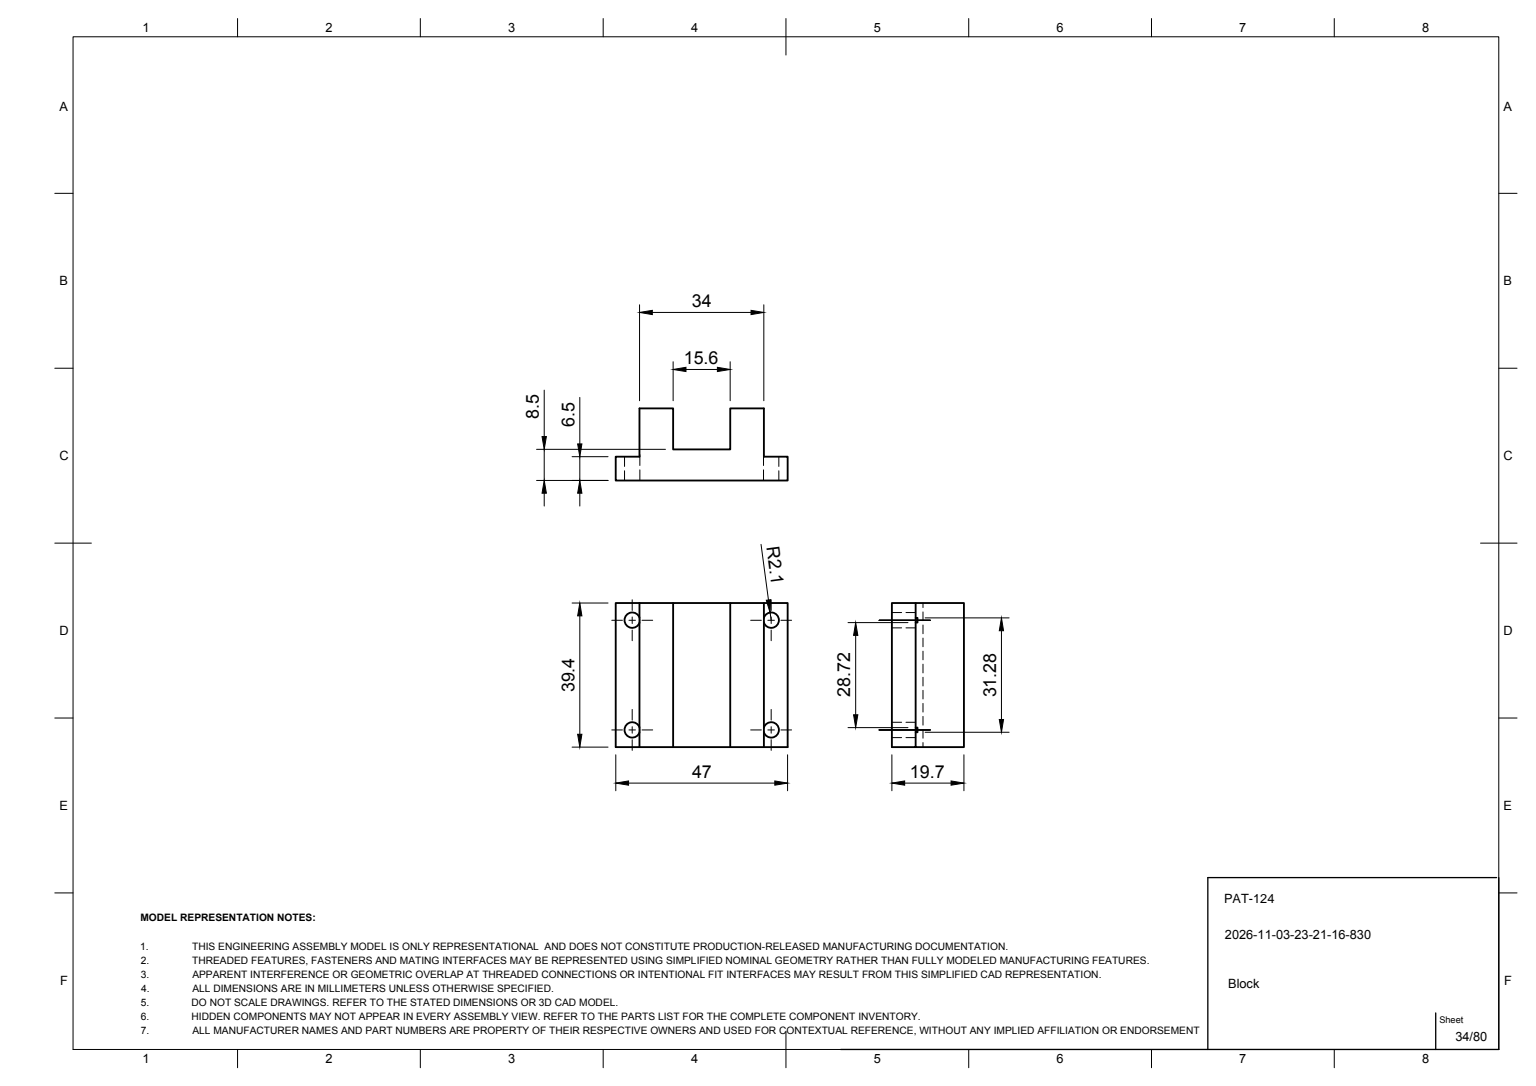
ISO-10303-21;
HEADER;
/* Generated by software containing ST-Developer
 * from STEP Tools, Inc. (www.steptools.com) 
 */

FILE_DESCRIPTION(
/* description */ ('XY cross-slide table'),
/* implementation_level */ '2;1');

FILE_NAME(
/* name */ 'Block.step',
/* time_stamp */ '2026-10-28T03:22:46-07:00',
/* author */ (''),
/* organization */ (''),
/* preprocessor_version */ 'ST-DEVELOPER v20.2',
/* originating_system */ 'Autodesk Translation Framework v15.17.0.0',
/* authorisation */ '');

FILE_SCHEMA (('AUTOMOTIVE_DESIGN { 1 0 10303 214 3 1 1 }'));
ENDSEC;

DATA;
#10=MECHANICAL_DESIGN_GEOMETRIC_PRESENTATION_REPRESENTATION('',(#1709),#62984);
#1528=SHAPE_REPRESENTATION_RELATIONSHIP('SRR','None',#63380,#1611);
#1611=ADVANCED_BREP_SHAPE_REPRESENTATION('',(#1822),#62917);
#1709=STYLED_ITEM('',(#63891),#1822);
#1822=MANIFOLD_SOLID_BREP('Body1',#23003);
#2042=FACE_BOUND('',#4647,.T.);
#2043=FACE_BOUND('',#4648,.T.);
#2044=FACE_BOUND('',#4649,.T.);
#2045=FACE_BOUND('',#4650,.T.);
#2439=PLANE('',#24650);
#2440=PLANE('',#24656);
#2441=PLANE('',#24662);
#2442=PLANE('',#24668);
#2443=PLANE('',#24674);
#2444=PLANE('',#24675);
#2445=PLANE('',#24676);
#2446=PLANE('',#24677);
#2447=PLANE('',#24678);
#2448=PLANE('',#24679);
#2449=PLANE('',#24680);
#2450=PLANE('',#24681);
#2451=PLANE('',#24682);
#2452=PLANE('',#24683);
#2453=PLANE('',#24684);
#2454=PLANE('',#24685);
#2455=PLANE('',#24686);
#2456=PLANE('',#24687);
#3164=FACE_OUTER_BOUND('',#4633,.T.);
#3165=FACE_OUTER_BOUND('',#4634,.T.);
#3166=FACE_OUTER_BOUND('',#4635,.T.);
#3167=FACE_OUTER_BOUND('',#4636,.T.);
#3168=FACE_OUTER_BOUND('',#4637,.T.);
#3169=FACE_OUTER_BOUND('',#4638,.T.);
#3170=FACE_OUTER_BOUND('',#4639,.T.);
#3171=FACE_OUTER_BOUND('',#4640,.T.);
#3172=FACE_OUTER_BOUND('',#4641,.T.);
#3173=FACE_OUTER_BOUND('',#4642,.T.);
#3174=FACE_OUTER_BOUND('',#4643,.T.);
#3175=FACE_OUTER_BOUND('',#4644,.T.);
#3176=FACE_OUTER_BOUND('',#4645,.T.);
#3177=FACE_OUTER_BOUND('',#4646,.T.);
#3178=FACE_OUTER_BOUND('',#4651,.T.);
#3179=FACE_OUTER_BOUND('',#4652,.T.);
#3180=FACE_OUTER_BOUND('',#4653,.T.);
#3181=FACE_OUTER_BOUND('',#4654,.T.);
#3182=FACE_OUTER_BOUND('',#4655,.T.);
#3183=FACE_OUTER_BOUND('',#4656,.T.);
#3184=FACE_OUTER_BOUND('',#4657,.T.);
#3185=FACE_OUTER_BOUND('',#4658,.T.);
#4633=EDGE_LOOP('',(#16180,#16181));
#4634=EDGE_LOOP('',(#16182,#16183,#16184,#16185,#16186,#16187,#16188,#16189));
#4635=EDGE_LOOP('',(#16190,#16191));
#4636=EDGE_LOOP('',(#16192,#16193,#16194,#16195,#16196,#16197,#16198,#16199));
#4637=EDGE_LOOP('',(#16200,#16201));
#4638=EDGE_LOOP('',(#16202,#16203,#16204,#16205,#16206,#16207,#16208,#16209));
#4639=EDGE_LOOP('',(#16210,#16211));
#4640=EDGE_LOOP('',(#16212,#16213,#16214,#16215,#16216,#16217,#16218,#16219));
#4641=EDGE_LOOP('',(#16220,#16221,#16222,#16223,#16224,#16225,#16226,#16227,
#16228,#16229,#16230,#16231));
#4642=EDGE_LOOP('',(#16232,#16233,#16234,#16235,#16236,#16237,#16238,#16239,
#16240,#16241,#16242,#16243));
#4643=EDGE_LOOP('',(#16244,#16245,#16246,#16247,#16248,#16249,#16250,#16251,
#16252,#16253,#16254,#16255));
#4644=EDGE_LOOP('',(#16256,#16257,#16258,#16259,#16260,#16261,#16262,#16263,
#16264,#16265));
#4645=EDGE_LOOP('',(#16266,#16267,#16268,#16269));
#4646=EDGE_LOOP('',(#16270,#16271,#16272,#16273));
#4647=EDGE_LOOP('',(#16274));
#4648=EDGE_LOOP('',(#16275));
#4649=EDGE_LOOP('',(#16276));
#4650=EDGE_LOOP('',(#16277));
#4651=EDGE_LOOP('',(#16278,#16279,#16280,#16281));
#4652=EDGE_LOOP('',(#16282,#16283,#16284,#16285,#16286,#16287,#16288,#16289,
#16290,#16291));
#4653=EDGE_LOOP('',(#16292,#16293,#16294,#16295));
#4654=EDGE_LOOP('',(#16296,#16297,#16298,#16299));
#4655=EDGE_LOOP('',(#16300,#16301,#16302,#16303));
#4656=EDGE_LOOP('',(#16304,#16305,#16306,#16307));
#4657=EDGE_LOOP('',(#16308,#16309,#16310,#16311));
#4658=EDGE_LOOP('',(#16312,#16313,#16314,#16315,#16316,#16317,#16318,#16319,
#16320,#16321,#16322,#16323));
#6199=LINE('',#34920,#7686);
#6200=LINE('',#34924,#7687);
#6201=LINE('',#34928,#7688);
#6202=LINE('',#34932,#7689);
#6203=LINE('',#34936,#7690);
#6204=LINE('',#34940,#7691);
#6205=LINE('',#34944,#7692);
#6206=LINE('',#34948,#7693);
#6207=LINE('',#34952,#7694);
#6208=LINE('',#34956,#7695);
#6209=LINE('',#34960,#7696);
#6210=LINE('',#34964,#7697);
#6211=LINE('',#34968,#7698);
#6212=LINE('',#34972,#7699);
#6213=LINE('',#34976,#7700);
#6214=LINE('',#34980,#7701);
#6215=LINE('',#34982,#7702);
#6216=LINE('',#34984,#7703);
#6217=LINE('',#34986,#7704);
#6218=LINE('',#34988,#7705);
#6219=LINE('',#34990,#7706);
#6220=LINE('',#34991,#7707);
#6221=LINE('',#34993,#7708);
#6222=LINE('',#34995,#7709);
#6223=LINE('',#34997,#7710);
#6224=LINE('',#34999,#7711);
#6225=LINE('',#35001,#7712);
#6226=LINE('',#35002,#7713);
#6227=LINE('',#35005,#7714);
#6228=LINE('',#35007,#7715);
#6229=LINE('',#35009,#7716);
#6230=LINE('',#35011,#7717);
#6231=LINE('',#35012,#7718);
#6232=LINE('',#35014,#7719);
#6233=LINE('',#35016,#7720);
#6234=LINE('',#35018,#7721);
#6235=LINE('',#35020,#7722);
#6236=LINE('',#35021,#7723);
#6237=LINE('',#35024,#7724);
#6238=LINE('',#35025,#7725);
#6239=LINE('',#35028,#7726);
#6240=LINE('',#35029,#7727);
#6241=LINE('',#35032,#7728);
#6242=LINE('',#35033,#7729);
#6243=LINE('',#35036,#7730);
#6244=LINE('',#35037,#7731);
#6245=LINE('',#35039,#7732);
#6246=LINE('',#35042,#7733);
#6247=LINE('',#35043,#7734);
#6248=LINE('',#35046,#7735);
#6249=LINE('',#35047,#7736);
#6250=LINE('',#35050,#7737);
#6251=LINE('',#35051,#7738);
#6252=LINE('',#35054,#7739);
#6253=LINE('',#35055,#7740);
#6254=LINE('',#35057,#7741);
#7686=VECTOR('',#28056,1.);
#7687=VECTOR('',#28061,1.);
#7688=VECTOR('',#28064,0.21);
#7689=VECTOR('',#28069,1.);
#7690=VECTOR('',#28072,1.);
#7691=VECTOR('',#28077,1.);
#7692=VECTOR('',#28080,0.21);
#7693=VECTOR('',#28085,1.);
#7694=VECTOR('',#28088,1.);
#7695=VECTOR('',#28093,1.);
#7696=VECTOR('',#28096,0.21);
#7697=VECTOR('',#28101,1.);
#7698=VECTOR('',#28104,1.);
#7699=VECTOR('',#28109,1.);
#7700=VECTOR('',#28112,0.21);
#7701=VECTOR('',#28117,1.);
#7702=VECTOR('',#28120,1.);
#7703=VECTOR('',#28121,1.);
#7704=VECTOR('',#28122,1.);
#7705=VECTOR('',#28123,1.);
#7706=VECTOR('',#28124,1.);
#7707=VECTOR('',#28125,1.);
#7708=VECTOR('',#28128,1.);
#7709=VECTOR('',#28129,1.);
#7710=VECTOR('',#28130,1.);
#7711=VECTOR('',#28131,1.);
#7712=VECTOR('',#28132,1.);
#7713=VECTOR('',#28133,1.);
#7714=VECTOR('',#28136,1.);
#7715=VECTOR('',#28137,1.);
#7716=VECTOR('',#28138,1.);
#7717=VECTOR('',#28139,1.);
#7718=VECTOR('',#28140,1.);
#7719=VECTOR('',#28141,1.);
#7720=VECTOR('',#28142,1.);
#7721=VECTOR('',#28143,1.);
#7722=VECTOR('',#28144,1.);
#7723=VECTOR('',#28145,1.);
#7724=VECTOR('',#28148,1.);
#7725=VECTOR('',#28149,1.);
#7726=VECTOR('',#28152,1.);
#7727=VECTOR('',#28153,1.);
#7728=VECTOR('',#28156,1.);
#7729=VECTOR('',#28157,1.);
#7730=VECTOR('',#28160,1.);
#7731=VECTOR('',#28161,1.);
#7732=VECTOR('',#28164,1.);
#7733=VECTOR('',#28167,1.);
#7734=VECTOR('',#28168,1.);
#7735=VECTOR('',#28171,1.);
#7736=VECTOR('',#28172,1.);
#7737=VECTOR('',#28175,1.);
#7738=VECTOR('',#28176,1.);
#7739=VECTOR('',#28179,1.);
#7740=VECTOR('',#28180,1.);
#7741=VECTOR('',#28183,1.);
#9193=CIRCLE('',#24651,0.21);
#9194=CIRCLE('',#24653,0.21);
#9195=CIRCLE('',#24654,0.21);
#9196=CIRCLE('',#24655,0.21);
#9197=CIRCLE('',#24657,0.21);
#9198=CIRCLE('',#24659,0.21);
#9199=CIRCLE('',#24660,0.21);
#9200=CIRCLE('',#24661,0.21);
#9201=CIRCLE('',#24663,0.21);
#9202=CIRCLE('',#24665,0.21);
#9203=CIRCLE('',#24666,0.21);
#9204=CIRCLE('',#24667,0.21);
#9205=CIRCLE('',#24669,0.21);
#9206=CIRCLE('',#24671,0.21);
#9207=CIRCLE('',#24672,0.21);
#9208=CIRCLE('',#24673,0.21);
#10213=VERTEX_POINT('',#34918);
#10214=VERTEX_POINT('',#34919);
#10215=VERTEX_POINT('',#34923);
#10216=VERTEX_POINT('',#34925);
#10217=VERTEX_POINT('',#34927);
#10218=VERTEX_POINT('',#34930);
#10219=VERTEX_POINT('',#34934);
#10220=VERTEX_POINT('',#34935);
#10221=VERTEX_POINT('',#34939);
#10222=VERTEX_POINT('',#34941);
#10223=VERTEX_POINT('',#34943);
#10224=VERTEX_POINT('',#34946);
#10225=VERTEX_POINT('',#34950);
#10226=VERTEX_POINT('',#34951);
#10227=VERTEX_POINT('',#34955);
#10228=VERTEX_POINT('',#34957);
#10229=VERTEX_POINT('',#34959);
#10230=VERTEX_POINT('',#34962);
#10231=VERTEX_POINT('',#34966);
#10232=VERTEX_POINT('',#34967);
#10233=VERTEX_POINT('',#34971);
#10234=VERTEX_POINT('',#34973);
#10235=VERTEX_POINT('',#34975);
#10236=VERTEX_POINT('',#34978);
#10237=VERTEX_POINT('',#34983);
#10238=VERTEX_POINT('',#34985);
#10239=VERTEX_POINT('',#34987);
#10240=VERTEX_POINT('',#34989);
#10241=VERTEX_POINT('',#34994);
#10242=VERTEX_POINT('',#34996);
#10243=VERTEX_POINT('',#34998);
#10244=VERTEX_POINT('',#35000);
#10245=VERTEX_POINT('',#35004);
#10246=VERTEX_POINT('',#35006);
#10247=VERTEX_POINT('',#35008);
#10248=VERTEX_POINT('',#35010);
#10249=VERTEX_POINT('',#35013);
#10250=VERTEX_POINT('',#35015);
#10251=VERTEX_POINT('',#35017);
#10252=VERTEX_POINT('',#35019);
#10253=VERTEX_POINT('',#35023);
#10254=VERTEX_POINT('',#35027);
#10255=VERTEX_POINT('',#35031);
#10256=VERTEX_POINT('',#35035);
#10257=VERTEX_POINT('',#35041);
#10258=VERTEX_POINT('',#35045);
#10259=VERTEX_POINT('',#35049);
#10260=VERTEX_POINT('',#35053);
#12474=EDGE_CURVE('',#10213,#10214,#6199,.T.);
#12475=EDGE_CURVE('',#10213,#10214,#9193,.T.);
#12476=EDGE_CURVE('',#10215,#10213,#6200,.T.);
#12477=EDGE_CURVE('',#10216,#10215,#9194,.T.);
#12478=EDGE_CURVE('',#10216,#10217,#6201,.T.);
#12479=EDGE_CURVE('',#10217,#10217,#9195,.T.);
#12480=EDGE_CURVE('',#10218,#10216,#9196,.T.);
#12481=EDGE_CURVE('',#10214,#10218,#6202,.T.);
#12482=EDGE_CURVE('',#10219,#10220,#6203,.T.);
#12483=EDGE_CURVE('',#10219,#10220,#9197,.T.);
#12484=EDGE_CURVE('',#10221,#10219,#6204,.T.);
#12485=EDGE_CURVE('',#10222,#10221,#9198,.T.);
#12486=EDGE_CURVE('',#10222,#10223,#6205,.T.);
#12487=EDGE_CURVE('',#10223,#10223,#9199,.T.);
#12488=EDGE_CURVE('',#10224,#10222,#9200,.T.);
#12489=EDGE_CURVE('',#10220,#10224,#6206,.T.);
#12490=EDGE_CURVE('',#10225,#10226,#6207,.T.);
#12491=EDGE_CURVE('',#10225,#10226,#9201,.T.);
#12492=EDGE_CURVE('',#10227,#10225,#6208,.T.);
#12493=EDGE_CURVE('',#10228,#10227,#9202,.T.);
#12494=EDGE_CURVE('',#10228,#10229,#6209,.T.);
#12495=EDGE_CURVE('',#10229,#10229,#9203,.T.);
#12496=EDGE_CURVE('',#10230,#10228,#9204,.T.);
#12497=EDGE_CURVE('',#10226,#10230,#6210,.T.);
#12498=EDGE_CURVE('',#10231,#10232,#6211,.T.);
#12499=EDGE_CURVE('',#10231,#10232,#9205,.T.);
#12500=EDGE_CURVE('',#10233,#10231,#6212,.T.);
#12501=EDGE_CURVE('',#10234,#10233,#9206,.T.);
#12502=EDGE_CURVE('',#10234,#10235,#6213,.T.);
#12503=EDGE_CURVE('',#10235,#10235,#9207,.T.);
#12504=EDGE_CURVE('',#10236,#10234,#9208,.T.);
#12505=EDGE_CURVE('',#10232,#10236,#6214,.T.);
#12506=EDGE_CURVE('',#10218,#10227,#6215,.T.);
#12507=EDGE_CURVE('',#10230,#10237,#6216,.T.);
#12508=EDGE_CURVE('',#10238,#10237,#6217,.T.);
#12509=EDGE_CURVE('',#10238,#10239,#6218,.T.);
#12510=EDGE_CURVE('',#10240,#10239,#6219,.T.);
#12511=EDGE_CURVE('',#10240,#10215,#6220,.T.);
#12512=EDGE_CURVE('',#10224,#10233,#6221,.T.);
#12513=EDGE_CURVE('',#10236,#10241,#6222,.T.);
#12514=EDGE_CURVE('',#10242,#10241,#6223,.T.);
#12515=EDGE_CURVE('',#10243,#10242,#6224,.T.);
#12516=EDGE_CURVE('',#10244,#10243,#6225,.T.);
#12517=EDGE_CURVE('',#10244,#10221,#6226,.T.);
#12518=EDGE_CURVE('',#10237,#10245,#6227,.T.);
#12519=EDGE_CURVE('',#10245,#10246,#6228,.T.);
#12520=EDGE_CURVE('',#10246,#10247,#6229,.T.);
#12521=EDGE_CURVE('',#10247,#10248,#6230,.T.);
#12522=EDGE_CURVE('',#10248,#10244,#6231,.T.);
#12523=EDGE_CURVE('',#10243,#10249,#6232,.T.);
#12524=EDGE_CURVE('',#10249,#10250,#6233,.T.);
#12525=EDGE_CURVE('',#10250,#10251,#6234,.T.);
#12526=EDGE_CURVE('',#10251,#10252,#6235,.T.);
#12527=EDGE_CURVE('',#10252,#10238,#6236,.T.);
#12528=EDGE_CURVE('',#10253,#10240,#6237,.T.);
#12529=EDGE_CURVE('',#10245,#10253,#6238,.T.);
#12530=EDGE_CURVE('',#10254,#10253,#6239,.T.);
#12531=EDGE_CURVE('',#10246,#10254,#6240,.T.);
#12532=EDGE_CURVE('',#10255,#10254,#6241,.T.);
#12533=EDGE_CURVE('',#10247,#10255,#6242,.T.);
#12534=EDGE_CURVE('',#10256,#10255,#6243,.T.);
#12535=EDGE_CURVE('',#10248,#10256,#6244,.T.);
#12536=EDGE_CURVE('',#10241,#10256,#6245,.T.);
#12537=EDGE_CURVE('',#10257,#10242,#6246,.T.);
#12538=EDGE_CURVE('',#10249,#10257,#6247,.T.);
#12539=EDGE_CURVE('',#10258,#10257,#6248,.T.);
#12540=EDGE_CURVE('',#10250,#10258,#6249,.T.);
#12541=EDGE_CURVE('',#10259,#10258,#6250,.T.);
#12542=EDGE_CURVE('',#10251,#10259,#6251,.T.);
#12543=EDGE_CURVE('',#10260,#10259,#6252,.T.);
#12544=EDGE_CURVE('',#10252,#10260,#6253,.T.);
#12545=EDGE_CURVE('',#10239,#10260,#6254,.T.);
#16180=ORIENTED_EDGE('',*,*,#12474,.F.);
#16181=ORIENTED_EDGE('',*,*,#12475,.T.);
#16182=ORIENTED_EDGE('',*,*,#12476,.F.);
#16183=ORIENTED_EDGE('',*,*,#12477,.F.);
#16184=ORIENTED_EDGE('',*,*,#12478,.T.);
#16185=ORIENTED_EDGE('',*,*,#12479,.F.);
#16186=ORIENTED_EDGE('',*,*,#12478,.F.);
#16187=ORIENTED_EDGE('',*,*,#12480,.F.);
#16188=ORIENTED_EDGE('',*,*,#12481,.F.);
#16189=ORIENTED_EDGE('',*,*,#12475,.F.);
#16190=ORIENTED_EDGE('',*,*,#12482,.F.);
#16191=ORIENTED_EDGE('',*,*,#12483,.T.);
#16192=ORIENTED_EDGE('',*,*,#12484,.F.);
#16193=ORIENTED_EDGE('',*,*,#12485,.F.);
#16194=ORIENTED_EDGE('',*,*,#12486,.T.);
#16195=ORIENTED_EDGE('',*,*,#12487,.F.);
#16196=ORIENTED_EDGE('',*,*,#12486,.F.);
#16197=ORIENTED_EDGE('',*,*,#12488,.F.);
#16198=ORIENTED_EDGE('',*,*,#12489,.F.);
#16199=ORIENTED_EDGE('',*,*,#12483,.F.);
#16200=ORIENTED_EDGE('',*,*,#12490,.F.);
#16201=ORIENTED_EDGE('',*,*,#12491,.T.);
#16202=ORIENTED_EDGE('',*,*,#12492,.F.);
#16203=ORIENTED_EDGE('',*,*,#12493,.F.);
#16204=ORIENTED_EDGE('',*,*,#12494,.T.);
#16205=ORIENTED_EDGE('',*,*,#12495,.F.);
#16206=ORIENTED_EDGE('',*,*,#12494,.F.);
#16207=ORIENTED_EDGE('',*,*,#12496,.F.);
#16208=ORIENTED_EDGE('',*,*,#12497,.F.);
#16209=ORIENTED_EDGE('',*,*,#12491,.F.);
#16210=ORIENTED_EDGE('',*,*,#12498,.F.);
#16211=ORIENTED_EDGE('',*,*,#12499,.T.);
#16212=ORIENTED_EDGE('',*,*,#12500,.F.);
#16213=ORIENTED_EDGE('',*,*,#12501,.F.);
#16214=ORIENTED_EDGE('',*,*,#12502,.T.);
#16215=ORIENTED_EDGE('',*,*,#12503,.F.);
#16216=ORIENTED_EDGE('',*,*,#12502,.F.);
#16217=ORIENTED_EDGE('',*,*,#12504,.F.);
#16218=ORIENTED_EDGE('',*,*,#12505,.F.);
#16219=ORIENTED_EDGE('',*,*,#12499,.F.);
#16220=ORIENTED_EDGE('',*,*,#12476,.T.);
#16221=ORIENTED_EDGE('',*,*,#12474,.T.);
#16222=ORIENTED_EDGE('',*,*,#12481,.T.);
#16223=ORIENTED_EDGE('',*,*,#12506,.T.);
#16224=ORIENTED_EDGE('',*,*,#12492,.T.);
#16225=ORIENTED_EDGE('',*,*,#12490,.T.);
#16226=ORIENTED_EDGE('',*,*,#12497,.T.);
#16227=ORIENTED_EDGE('',*,*,#12507,.T.);
#16228=ORIENTED_EDGE('',*,*,#12508,.F.);
#16229=ORIENTED_EDGE('',*,*,#12509,.T.);
#16230=ORIENTED_EDGE('',*,*,#12510,.F.);
#16231=ORIENTED_EDGE('',*,*,#12511,.T.);
#16232=ORIENTED_EDGE('',*,*,#12484,.T.);
#16233=ORIENTED_EDGE('',*,*,#12482,.T.);
#16234=ORIENTED_EDGE('',*,*,#12489,.T.);
#16235=ORIENTED_EDGE('',*,*,#12512,.T.);
#16236=ORIENTED_EDGE('',*,*,#12500,.T.);
#16237=ORIENTED_EDGE('',*,*,#12498,.T.);
#16238=ORIENTED_EDGE('',*,*,#12505,.T.);
#16239=ORIENTED_EDGE('',*,*,#12513,.T.);
#16240=ORIENTED_EDGE('',*,*,#12514,.F.);
#16241=ORIENTED_EDGE('',*,*,#12515,.F.);
#16242=ORIENTED_EDGE('',*,*,#12516,.F.);
#16243=ORIENTED_EDGE('',*,*,#12517,.T.);
#16244=ORIENTED_EDGE('',*,*,#12508,.T.);
#16245=ORIENTED_EDGE('',*,*,#12518,.T.);
#16246=ORIENTED_EDGE('',*,*,#12519,.T.);
#16247=ORIENTED_EDGE('',*,*,#12520,.T.);
#16248=ORIENTED_EDGE('',*,*,#12521,.T.);
#16249=ORIENTED_EDGE('',*,*,#12522,.T.);
#16250=ORIENTED_EDGE('',*,*,#12516,.T.);
#16251=ORIENTED_EDGE('',*,*,#12523,.T.);
#16252=ORIENTED_EDGE('',*,*,#12524,.T.);
#16253=ORIENTED_EDGE('',*,*,#12525,.T.);
#16254=ORIENTED_EDGE('',*,*,#12526,.T.);
#16255=ORIENTED_EDGE('',*,*,#12527,.T.);
#16256=ORIENTED_EDGE('',*,*,#12480,.T.);
#16257=ORIENTED_EDGE('',*,*,#12477,.T.);
#16258=ORIENTED_EDGE('',*,*,#12511,.F.);
#16259=ORIENTED_EDGE('',*,*,#12528,.F.);
#16260=ORIENTED_EDGE('',*,*,#12529,.F.);
#16261=ORIENTED_EDGE('',*,*,#12518,.F.);
#16262=ORIENTED_EDGE('',*,*,#12507,.F.);
#16263=ORIENTED_EDGE('',*,*,#12496,.T.);
#16264=ORIENTED_EDGE('',*,*,#12493,.T.);
#16265=ORIENTED_EDGE('',*,*,#12506,.F.);
#16266=ORIENTED_EDGE('',*,*,#12529,.T.);
#16267=ORIENTED_EDGE('',*,*,#12530,.F.);
#16268=ORIENTED_EDGE('',*,*,#12531,.F.);
#16269=ORIENTED_EDGE('',*,*,#12519,.F.);
#16270=ORIENTED_EDGE('',*,*,#12531,.T.);
#16271=ORIENTED_EDGE('',*,*,#12532,.F.);
#16272=ORIENTED_EDGE('',*,*,#12533,.F.);
#16273=ORIENTED_EDGE('',*,*,#12520,.F.);
#16274=ORIENTED_EDGE('',*,*,#12479,.T.);
#16275=ORIENTED_EDGE('',*,*,#12487,.T.);
#16276=ORIENTED_EDGE('',*,*,#12495,.T.);
#16277=ORIENTED_EDGE('',*,*,#12503,.T.);
#16278=ORIENTED_EDGE('',*,*,#12533,.T.);
#16279=ORIENTED_EDGE('',*,*,#12534,.F.);
#16280=ORIENTED_EDGE('',*,*,#12535,.F.);
#16281=ORIENTED_EDGE('',*,*,#12521,.F.);
#16282=ORIENTED_EDGE('',*,*,#12488,.T.);
#16283=ORIENTED_EDGE('',*,*,#12485,.T.);
#16284=ORIENTED_EDGE('',*,*,#12517,.F.);
#16285=ORIENTED_EDGE('',*,*,#12522,.F.);
#16286=ORIENTED_EDGE('',*,*,#12535,.T.);
#16287=ORIENTED_EDGE('',*,*,#12536,.F.);
#16288=ORIENTED_EDGE('',*,*,#12513,.F.);
#16289=ORIENTED_EDGE('',*,*,#12504,.T.);
#16290=ORIENTED_EDGE('',*,*,#12501,.T.);
#16291=ORIENTED_EDGE('',*,*,#12512,.F.);
#16292=ORIENTED_EDGE('',*,*,#12515,.T.);
#16293=ORIENTED_EDGE('',*,*,#12537,.F.);
#16294=ORIENTED_EDGE('',*,*,#12538,.F.);
#16295=ORIENTED_EDGE('',*,*,#12523,.F.);
#16296=ORIENTED_EDGE('',*,*,#12538,.T.);
#16297=ORIENTED_EDGE('',*,*,#12539,.F.);
#16298=ORIENTED_EDGE('',*,*,#12540,.F.);
#16299=ORIENTED_EDGE('',*,*,#12524,.F.);
#16300=ORIENTED_EDGE('',*,*,#12540,.T.);
#16301=ORIENTED_EDGE('',*,*,#12541,.F.);
#16302=ORIENTED_EDGE('',*,*,#12542,.F.);
#16303=ORIENTED_EDGE('',*,*,#12525,.F.);
#16304=ORIENTED_EDGE('',*,*,#12542,.T.);
#16305=ORIENTED_EDGE('',*,*,#12543,.F.);
#16306=ORIENTED_EDGE('',*,*,#12544,.F.);
#16307=ORIENTED_EDGE('',*,*,#12526,.F.);
#16308=ORIENTED_EDGE('',*,*,#12544,.T.);
#16309=ORIENTED_EDGE('',*,*,#12545,.F.);
#16310=ORIENTED_EDGE('',*,*,#12509,.F.);
#16311=ORIENTED_EDGE('',*,*,#12527,.F.);
#16312=ORIENTED_EDGE('',*,*,#12510,.T.);
#16313=ORIENTED_EDGE('',*,*,#12545,.T.);
#16314=ORIENTED_EDGE('',*,*,#12543,.T.);
#16315=ORIENTED_EDGE('',*,*,#12541,.T.);
#16316=ORIENTED_EDGE('',*,*,#12539,.T.);
#16317=ORIENTED_EDGE('',*,*,#12537,.T.);
#16318=ORIENTED_EDGE('',*,*,#12514,.T.);
#16319=ORIENTED_EDGE('',*,*,#12536,.T.);
#16320=ORIENTED_EDGE('',*,*,#12534,.T.);
#16321=ORIENTED_EDGE('',*,*,#12532,.T.);
#16322=ORIENTED_EDGE('',*,*,#12530,.T.);
#16323=ORIENTED_EDGE('',*,*,#12528,.T.);
#21150=CYLINDRICAL_SURFACE('',#24652,0.21);
#21151=CYLINDRICAL_SURFACE('',#24658,0.21);
#21152=CYLINDRICAL_SURFACE('',#24664,0.21);
#21153=CYLINDRICAL_SURFACE('',#24670,0.21);
#21945=ADVANCED_FACE('',(#3164),#2439,.T.);
#21946=ADVANCED_FACE('',(#3165),#21150,.F.);
#21947=ADVANCED_FACE('',(#3166),#2440,.T.);
#21948=ADVANCED_FACE('',(#3167),#21151,.F.);
#21949=ADVANCED_FACE('',(#3168),#2441,.T.);
#21950=ADVANCED_FACE('',(#3169),#21152,.F.);
#21951=ADVANCED_FACE('',(#3170),#2442,.T.);
#21952=ADVANCED_FACE('',(#3171),#21153,.F.);
#21953=ADVANCED_FACE('',(#3172),#2443,.T.);
#21954=ADVANCED_FACE('',(#3173),#2444,.T.);
#21955=ADVANCED_FACE('',(#3174),#2445,.T.);
#21956=ADVANCED_FACE('',(#3175),#2446,.T.);
#21957=ADVANCED_FACE('',(#3176),#2447,.T.);
#21958=ADVANCED_FACE('',(#3177,#2042,#2043,#2044,#2045),#2448,.T.);
#21959=ADVANCED_FACE('',(#3178),#2449,.T.);
#21960=ADVANCED_FACE('',(#3179),#2450,.T.);
#21961=ADVANCED_FACE('',(#3180),#2451,.T.);
#21962=ADVANCED_FACE('',(#3181),#2452,.T.);
#21963=ADVANCED_FACE('',(#3182),#2453,.T.);
#21964=ADVANCED_FACE('',(#3183),#2454,.T.);
#21965=ADVANCED_FACE('',(#3184),#2455,.T.);
#21966=ADVANCED_FACE('',(#3185),#2456,.T.);
#23003=CLOSED_SHELL('',(#21945,#21946,#21947,#21948,#21949,#21950,#21951,
#21952,#21953,#21954,#21955,#21956,#21957,#21958,#21959,#21960,#21961,#21962,
#21963,#21964,#21965,#21966));
#24649=AXIS2_PLACEMENT_3D('',#34916,#28052,#28053);
#24650=AXIS2_PLACEMENT_3D('',#34917,#28054,#28055);
#24651=AXIS2_PLACEMENT_3D('',#34921,#28057,#28058);
#24652=AXIS2_PLACEMENT_3D('',#34922,#28059,#28060);
#24653=AXIS2_PLACEMENT_3D('',#34926,#28062,#28063);
#24654=AXIS2_PLACEMENT_3D('',#34929,#28065,#28066);
#24655=AXIS2_PLACEMENT_3D('',#34931,#28067,#28068);
#24656=AXIS2_PLACEMENT_3D('',#34933,#28070,#28071);
#24657=AXIS2_PLACEMENT_3D('',#34937,#28073,#28074);
#24658=AXIS2_PLACEMENT_3D('',#34938,#28075,#28076);
#24659=AXIS2_PLACEMENT_3D('',#34942,#28078,#28079);
#24660=AXIS2_PLACEMENT_3D('',#34945,#28081,#28082);
#24661=AXIS2_PLACEMENT_3D('',#34947,#28083,#28084);
#24662=AXIS2_PLACEMENT_3D('',#34949,#28086,#28087);
#24663=AXIS2_PLACEMENT_3D('',#34953,#28089,#28090);
#24664=AXIS2_PLACEMENT_3D('',#34954,#28091,#28092);
#24665=AXIS2_PLACEMENT_3D('',#34958,#28094,#28095);
#24666=AXIS2_PLACEMENT_3D('',#34961,#28097,#28098);
#24667=AXIS2_PLACEMENT_3D('',#34963,#28099,#28100);
#24668=AXIS2_PLACEMENT_3D('',#34965,#28102,#28103);
#24669=AXIS2_PLACEMENT_3D('',#34969,#28105,#28106);
#24670=AXIS2_PLACEMENT_3D('',#34970,#28107,#28108);
#24671=AXIS2_PLACEMENT_3D('',#34974,#28110,#28111);
#24672=AXIS2_PLACEMENT_3D('',#34977,#28113,#28114);
#24673=AXIS2_PLACEMENT_3D('',#34979,#28115,#28116);
#24674=AXIS2_PLACEMENT_3D('',#34981,#28118,#28119);
#24675=AXIS2_PLACEMENT_3D('',#34992,#28126,#28127);
#24676=AXIS2_PLACEMENT_3D('',#35003,#28134,#28135);
#24677=AXIS2_PLACEMENT_3D('',#35022,#28146,#28147);
#24678=AXIS2_PLACEMENT_3D('',#35026,#28150,#28151);
#24679=AXIS2_PLACEMENT_3D('',#35030,#28154,#28155);
#24680=AXIS2_PLACEMENT_3D('',#35034,#28158,#28159);
#24681=AXIS2_PLACEMENT_3D('',#35038,#28162,#28163);
#24682=AXIS2_PLACEMENT_3D('',#35040,#28165,#28166);
#24683=AXIS2_PLACEMENT_3D('',#35044,#28169,#28170);
#24684=AXIS2_PLACEMENT_3D('',#35048,#28173,#28174);
#24685=AXIS2_PLACEMENT_3D('',#35052,#28177,#28178);
#24686=AXIS2_PLACEMENT_3D('',#35056,#28181,#28182);
#24687=AXIS2_PLACEMENT_3D('',#35058,#28184,#28185);
#28052=DIRECTION('axis',(0.,0.,1.));
#28053=DIRECTION('refdir',(1.,0.,0.));
#28054=DIRECTION('center_axis',(0.,0.,1.));
#28055=DIRECTION('ref_axis',(1.,0.,0.));
#28056=DIRECTION('',(-1.,0.,0.));
#28057=DIRECTION('center_axis',(0.,0.,1.));
#28058=DIRECTION('ref_axis',(1.,0.,0.));
#28059=DIRECTION('center_axis',(0.,0.,1.));
#28060=DIRECTION('ref_axis',(1.,0.,0.));
#28061=DIRECTION('',(0.,0.,-1.));
#28062=DIRECTION('center_axis',(0.,0.,1.));
#28063=DIRECTION('ref_axis',(1.,0.,0.));
#28064=DIRECTION('',(0.,0.,1.));
#28065=DIRECTION('center_axis',(0.,0.,-1.));
#28066=DIRECTION('ref_axis',(1.,0.,0.));
#28067=DIRECTION('center_axis',(0.,0.,1.));
#28068=DIRECTION('ref_axis',(1.,0.,0.));
#28069=DIRECTION('',(0.,0.,1.));
#28070=DIRECTION('center_axis',(0.,0.,1.));
#28071=DIRECTION('ref_axis',(1.,0.,0.));
#28072=DIRECTION('',(1.,0.,0.));
#28073=DIRECTION('center_axis',(0.,0.,1.));
#28074=DIRECTION('ref_axis',(1.,0.,0.));
#28075=DIRECTION('center_axis',(0.,0.,1.));
#28076=DIRECTION('ref_axis',(1.,0.,0.));
#28077=DIRECTION('',(0.,0.,-1.));
#28078=DIRECTION('center_axis',(0.,0.,1.));
#28079=DIRECTION('ref_axis',(1.,0.,0.));
#28080=DIRECTION('',(0.,0.,1.));
#28081=DIRECTION('center_axis',(0.,0.,-1.));
#28082=DIRECTION('ref_axis',(1.,0.,0.));
#28083=DIRECTION('center_axis',(0.,0.,1.));
#28084=DIRECTION('ref_axis',(1.,0.,0.));
#28085=DIRECTION('',(0.,0.,1.));
#28086=DIRECTION('center_axis',(0.,0.,1.));
#28087=DIRECTION('ref_axis',(1.,0.,0.));
#28088=DIRECTION('',(-1.,0.,0.));
#28089=DIRECTION('center_axis',(0.,0.,1.));
#28090=DIRECTION('ref_axis',(1.,0.,0.));
#28091=DIRECTION('center_axis',(0.,0.,1.));
#28092=DIRECTION('ref_axis',(1.,0.,0.));
#28093=DIRECTION('',(0.,0.,-1.));
#28094=DIRECTION('center_axis',(0.,0.,1.));
#28095=DIRECTION('ref_axis',(1.,0.,0.));
#28096=DIRECTION('',(0.,0.,1.));
#28097=DIRECTION('center_axis',(0.,0.,-1.));
#28098=DIRECTION('ref_axis',(1.,0.,0.));
#28099=DIRECTION('center_axis',(0.,0.,1.));
#28100=DIRECTION('ref_axis',(1.,0.,0.));
#28101=DIRECTION('',(0.,0.,1.));
#28102=DIRECTION('center_axis',(0.,0.,1.));
#28103=DIRECTION('ref_axis',(1.,0.,0.));
#28104=DIRECTION('',(1.,0.,0.));
#28105=DIRECTION('center_axis',(0.,0.,1.));
#28106=DIRECTION('ref_axis',(1.,0.,0.));
#28107=DIRECTION('center_axis',(0.,0.,1.));
#28108=DIRECTION('ref_axis',(1.,0.,0.));
#28109=DIRECTION('',(0.,0.,-1.));
#28110=DIRECTION('center_axis',(0.,0.,1.));
#28111=DIRECTION('ref_axis',(1.,0.,0.));
#28112=DIRECTION('',(0.,0.,1.));
#28113=DIRECTION('center_axis',(0.,0.,-1.));
#28114=DIRECTION('ref_axis',(1.,0.,0.));
#28115=DIRECTION('center_axis',(0.,0.,1.));
#28116=DIRECTION('ref_axis',(1.,0.,0.));
#28117=DIRECTION('',(0.,0.,1.));
#28118=DIRECTION('center_axis',(0.,-1.,0.));
#28119=DIRECTION('ref_axis',(0.,0.,-1.));
#28120=DIRECTION('',(-1.,0.,0.));
#28121=DIRECTION('',(-1.,0.,0.));
#28122=DIRECTION('',(0.,0.,1.));
#28123=DIRECTION('',(1.,0.,0.));
#28124=DIRECTION('',(0.,0.,-1.));
#28125=DIRECTION('',(-1.,0.,0.));
#28126=DIRECTION('center_axis',(0.,1.,0.));
#28127=DIRECTION('ref_axis',(0.,0.,1.));
#28128=DIRECTION('',(1.,0.,0.));
#28129=DIRECTION('',(1.,0.,0.));
#28130=DIRECTION('',(0.,0.,1.));
#28131=DIRECTION('',(1.,0.,0.));
#28132=DIRECTION('',(0.,0.,-1.));
#28133=DIRECTION('',(1.,0.,0.));
#28134=DIRECTION('center_axis',(-1.,0.,0.));
#28135=DIRECTION('ref_axis',(0.,0.,1.));
#28136=DIRECTION('',(0.,-1.,0.));
#28137=DIRECTION('',(0.,0.,1.));
#28138=DIRECTION('',(0.,1.,0.));
#28139=DIRECTION('',(0.,0.,-1.));
#28140=DIRECTION('',(0.,-1.,0.));
#28141=DIRECTION('',(0.,-1.,0.));
#28142=DIRECTION('',(0.,0.,1.));
#28143=DIRECTION('',(0.,-1.,0.));
#28144=DIRECTION('',(0.,0.,-1.));
#28145=DIRECTION('',(0.,-1.,0.));
#28146=DIRECTION('center_axis',(0.,0.,-1.));
#28147=DIRECTION('ref_axis',(0.,1.,0.));
#28148=DIRECTION('',(0.,1.,0.));
#28149=DIRECTION('',(1.,0.,0.));
#28150=DIRECTION('center_axis',(0.,-1.,0.));
#28151=DIRECTION('ref_axis',(0.,0.,-1.));
#28152=DIRECTION('',(0.,0.,-1.));
#28153=DIRECTION('',(1.,0.,0.));
#28154=DIRECTION('center_axis',(0.,0.,1.));
#28155=DIRECTION('ref_axis',(0.,-1.,0.));
#28156=DIRECTION('',(0.,-1.,0.));
#28157=DIRECTION('',(1.,0.,0.));
#28158=DIRECTION('center_axis',(0.,1.,0.));
#28159=DIRECTION('ref_axis',(0.,0.,1.));
#28160=DIRECTION('',(0.,0.,1.));
#28161=DIRECTION('',(1.,0.,0.));
#28162=DIRECTION('center_axis',(0.,0.,-1.));
#28163=DIRECTION('ref_axis',(0.,1.,0.));
#28164=DIRECTION('',(0.,1.,0.));
#28165=DIRECTION('center_axis',(0.,0.,-1.));
#28166=DIRECTION('ref_axis',(0.,1.,0.));
#28167=DIRECTION('',(0.,1.,0.));
#28168=DIRECTION('',(1.,0.,0.));
#28169=DIRECTION('center_axis',(0.,-1.,0.));
#28170=DIRECTION('ref_axis',(0.,0.,-1.));
#28171=DIRECTION('',(0.,0.,-1.));
#28172=DIRECTION('',(1.,0.,0.));
#28173=DIRECTION('center_axis',(0.,0.,-1.));
#28174=DIRECTION('ref_axis',(0.,1.,0.));
#28175=DIRECTION('',(0.,1.,0.));
#28176=DIRECTION('',(1.,0.,0.));
#28177=DIRECTION('center_axis',(0.,1.,0.));
#28178=DIRECTION('ref_axis',(0.,0.,1.));
#28179=DIRECTION('',(0.,0.,1.));
#28180=DIRECTION('',(1.,0.,0.));
#28181=DIRECTION('center_axis',(0.,0.,-1.));
#28182=DIRECTION('ref_axis',(0.,1.,0.));
#28183=DIRECTION('',(0.,1.,0.));
#28184=DIRECTION('center_axis',(1.,0.,0.));
#28185=DIRECTION('ref_axis',(0.,0.,-1.));
#34916=CARTESIAN_POINT('',(0.,0.,0.));
#34917=CARTESIAN_POINT('Origin',(1.5,-1.9,1.7));
#34918=CARTESIAN_POINT('',(1.56403124237433,-1.7,1.7));
#34919=CARTESIAN_POINT('',(1.43596875762567,-1.7,1.7));
#34920=CARTESIAN_POINT('',(0.75,-1.7,1.7));
#34921=CARTESIAN_POINT('Origin',(1.5,-1.9,1.7));
#34922=CARTESIAN_POINT('Origin',(1.5,-1.9,1.7));
#34923=CARTESIAN_POINT('',(1.56403124237433,-1.7,1.75));
#34924=CARTESIAN_POINT('',(1.56403124237433,-1.7,1.7));
#34925=CARTESIAN_POINT('',(1.29,-1.9,1.75));
#34926=CARTESIAN_POINT('Origin',(1.5,-1.9,1.75));
#34927=CARTESIAN_POINT('',(1.29,-1.9,2.4));
#34928=CARTESIAN_POINT('',(1.29,-1.9,1.7));
#34929=CARTESIAN_POINT('Origin',(1.5,-1.9,2.4));
#34930=CARTESIAN_POINT('',(1.43596875762567,-1.7,1.75));
#34931=CARTESIAN_POINT('Origin',(1.5,-1.9,1.75));
#34932=CARTESIAN_POINT('',(1.43596875762567,-1.7,1.7));
#34933=CARTESIAN_POINT('Origin',(-1.5,1.9,1.7));
#34934=CARTESIAN_POINT('',(-1.56403124237433,1.7,1.7));
#34935=CARTESIAN_POINT('',(-1.43596875762567,1.7,1.7));
#34936=CARTESIAN_POINT('',(-0.75,1.7,1.7));
#34937=CARTESIAN_POINT('Origin',(-1.5,1.9,1.7));
#34938=CARTESIAN_POINT('Origin',(-1.5,1.9,1.7));
#34939=CARTESIAN_POINT('',(-1.56403124237433,1.7,1.75));
#34940=CARTESIAN_POINT('',(-1.56403124237433,1.7,1.7));
#34941=CARTESIAN_POINT('',(-1.71,1.9,1.75));
#34942=CARTESIAN_POINT('Origin',(-1.5,1.9,1.75));
#34943=CARTESIAN_POINT('',(-1.71,1.9,2.4));
#34944=CARTESIAN_POINT('',(-1.71,1.9,1.7));
#34945=CARTESIAN_POINT('Origin',(-1.5,1.9,2.4));
#34946=CARTESIAN_POINT('',(-1.43596875762567,1.7,1.75));
#34947=CARTESIAN_POINT('Origin',(-1.5,1.9,1.75));
#34948=CARTESIAN_POINT('',(-1.43596875762567,1.7,1.7));
#34949=CARTESIAN_POINT('Origin',(-1.5,-1.9,1.7));
#34950=CARTESIAN_POINT('',(-1.43596875762567,-1.7,1.7));
#34951=CARTESIAN_POINT('',(-1.56403124237433,-1.7,1.7));
#34952=CARTESIAN_POINT('',(-0.75,-1.7,1.7));
#34953=CARTESIAN_POINT('Origin',(-1.5,-1.9,1.7));
#34954=CARTESIAN_POINT('Origin',(-1.5,-1.9,1.7));
#34955=CARTESIAN_POINT('',(-1.43596875762567,-1.7,1.75));
#34956=CARTESIAN_POINT('',(-1.43596875762567,-1.7,1.7));
#34957=CARTESIAN_POINT('',(-1.71,-1.9,1.75));
#34958=CARTESIAN_POINT('Origin',(-1.5,-1.9,1.75));
#34959=CARTESIAN_POINT('',(-1.71,-1.9,2.4));
#34960=CARTESIAN_POINT('',(-1.71,-1.9,1.7));
#34961=CARTESIAN_POINT('Origin',(-1.5,-1.9,2.4));
#34962=CARTESIAN_POINT('',(-1.56403124237433,-1.7,1.75));
#34963=CARTESIAN_POINT('Origin',(-1.5,-1.9,1.75));
#34964=CARTESIAN_POINT('',(-1.56403124237433,-1.7,1.7));
#34965=CARTESIAN_POINT('Origin',(1.5,1.9,1.7));
#34966=CARTESIAN_POINT('',(1.43596875762567,1.7,1.7));
#34967=CARTESIAN_POINT('',(1.56403124237433,1.7,1.7));
#34968=CARTESIAN_POINT('',(0.75,1.7,1.7));
#34969=CARTESIAN_POINT('Origin',(1.5,1.9,1.7));
#34970=CARTESIAN_POINT('Origin',(1.5,1.9,1.7));
#34971=CARTESIAN_POINT('',(1.43596875762567,1.7,1.75));
#34972=CARTESIAN_POINT('',(1.43596875762567,1.7,1.7));
#34973=CARTESIAN_POINT('',(1.29,1.9,1.75));
#34974=CARTESIAN_POINT('Origin',(1.5,1.9,1.75));
#34975=CARTESIAN_POINT('',(1.29,1.9,2.4));
#34976=CARTESIAN_POINT('',(1.29,1.9,1.7));
#34977=CARTESIAN_POINT('Origin',(1.5,1.9,2.4));
#34978=CARTESIAN_POINT('',(1.56403124237433,1.7,1.75));
#34979=CARTESIAN_POINT('Origin',(1.5,1.9,1.75));
#34980=CARTESIAN_POINT('',(1.56403124237433,1.7,1.7));
#34981=CARTESIAN_POINT('Origin',(0.,-1.7,1.75));
#34982=CARTESIAN_POINT('',(0.,-1.7,1.75));
#34983=CARTESIAN_POINT('',(-1.97,-1.7,1.75));
#34984=CARTESIAN_POINT('',(0.,-1.7,1.75));
#34985=CARTESIAN_POINT('',(-1.97,-1.7,0.43));
#34986=CARTESIAN_POINT('',(-1.97,-1.7,1.75));
#34987=CARTESIAN_POINT('',(1.97,-1.7,0.43));
#34988=CARTESIAN_POINT('',(0.,-1.7,0.43));
#34989=CARTESIAN_POINT('',(1.97,-1.7,1.75));
#34990=CARTESIAN_POINT('',(1.97,-1.7,1.75));
#34991=CARTESIAN_POINT('',(0.,-1.7,1.75));
#34992=CARTESIAN_POINT('Origin',(0.,1.7,0.43));
#34993=CARTESIAN_POINT('',(0.,1.7,1.75));
#34994=CARTESIAN_POINT('',(1.97,1.7,1.75));
#34995=CARTESIAN_POINT('',(0.,1.7,1.75));
#34996=CARTESIAN_POINT('',(1.97,1.7,0.43));
#34997=CARTESIAN_POINT('',(1.97,1.7,0.43));
#34998=CARTESIAN_POINT('',(-1.97,1.7,0.43));
#34999=CARTESIAN_POINT('',(0.,1.7,0.43));
#35000=CARTESIAN_POINT('',(-1.97,1.7,1.75));
#35001=CARTESIAN_POINT('',(-1.97,1.7,0.43));
#35002=CARTESIAN_POINT('',(0.,1.7,1.75));
#35003=CARTESIAN_POINT('Origin',(-1.97,0.,1.415));
#35004=CARTESIAN_POINT('',(-1.97,-2.35,1.75));
#35005=CARTESIAN_POINT('',(-1.97,-2.35,1.75));
#35006=CARTESIAN_POINT('',(-1.97,-2.35,2.4));
#35007=CARTESIAN_POINT('',(-1.97,-2.35,2.4));
#35008=CARTESIAN_POINT('',(-1.97,2.35,2.4));
#35009=CARTESIAN_POINT('',(-1.97,2.35,2.4));
#35010=CARTESIAN_POINT('',(-1.97,2.35,1.75));
#35011=CARTESIAN_POINT('',(-1.97,2.35,1.75));
#35012=CARTESIAN_POINT('',(-1.97,1.7,1.75));
#35013=CARTESIAN_POINT('',(-1.97,0.78,0.43));
#35014=CARTESIAN_POINT('',(-1.97,0.78,0.43));
#35015=CARTESIAN_POINT('',(-1.97,0.78,1.55));
#35016=CARTESIAN_POINT('',(-1.97,0.78,1.55));
#35017=CARTESIAN_POINT('',(-1.97,-0.78,1.55));
#35018=CARTESIAN_POINT('',(-1.97,-0.78,1.55));
#35019=CARTESIAN_POINT('',(-1.97,-0.78,0.43));
#35020=CARTESIAN_POINT('',(-1.97,-0.78,0.43));
#35021=CARTESIAN_POINT('',(-1.97,-1.7,0.43));
#35022=CARTESIAN_POINT('Origin',(0.,-2.35,1.75));
#35023=CARTESIAN_POINT('',(1.97,-2.35,1.75));
#35024=CARTESIAN_POINT('',(1.97,-2.35,1.75));
#35025=CARTESIAN_POINT('',(0.,-2.35,1.75));
#35026=CARTESIAN_POINT('Origin',(0.,-2.35,2.4));
#35027=CARTESIAN_POINT('',(1.97,-2.35,2.4));
#35028=CARTESIAN_POINT('',(1.97,-2.35,2.4));
#35029=CARTESIAN_POINT('',(0.,-2.35,2.4));
#35030=CARTESIAN_POINT('Origin',(0.,2.35,2.4));
#35031=CARTESIAN_POINT('',(1.97,2.35,2.4));
#35032=CARTESIAN_POINT('',(1.97,2.35,2.4));
#35033=CARTESIAN_POINT('',(0.,2.35,2.4));
#35034=CARTESIAN_POINT('Origin',(0.,2.35,1.75));
#35035=CARTESIAN_POINT('',(1.97,2.35,1.75));
#35036=CARTESIAN_POINT('',(1.97,2.35,1.75));
#35037=CARTESIAN_POINT('',(0.,2.35,1.75));
#35038=CARTESIAN_POINT('Origin',(0.,1.7,1.75));
#35039=CARTESIAN_POINT('',(1.97,1.7,1.75));
#35040=CARTESIAN_POINT('Origin',(0.,0.78,0.43));
#35041=CARTESIAN_POINT('',(1.97,0.78,0.43));
#35042=CARTESIAN_POINT('',(1.97,0.78,0.43));
#35043=CARTESIAN_POINT('',(0.,0.78,0.43));
#35044=CARTESIAN_POINT('Origin',(0.,0.78,1.55));
#35045=CARTESIAN_POINT('',(1.97,0.78,1.55));
#35046=CARTESIAN_POINT('',(1.97,0.78,1.55));
#35047=CARTESIAN_POINT('',(0.,0.78,1.55));
#35048=CARTESIAN_POINT('Origin',(0.,-0.78,1.55));
#35049=CARTESIAN_POINT('',(1.97,-0.78,1.55));
#35050=CARTESIAN_POINT('',(1.97,-0.78,1.55));
#35051=CARTESIAN_POINT('',(0.,-0.78,1.55));
#35052=CARTESIAN_POINT('Origin',(0.,-0.78,0.43));
#35053=CARTESIAN_POINT('',(1.97,-0.78,0.43));
#35054=CARTESIAN_POINT('',(1.97,-0.78,0.43));
#35055=CARTESIAN_POINT('',(0.,-0.78,0.43));
#35056=CARTESIAN_POINT('Origin',(0.,-1.7,0.43));
#35057=CARTESIAN_POINT('',(1.97,-1.7,0.43));
#35058=CARTESIAN_POINT('Origin',(1.97,0.,1.415));
#62818=UNCERTAINTY_MEASURE_WITH_UNIT(LENGTH_MEASURE(0.001),#62985,
'DISTANCE_ACCURACY_VALUE',
'Maximum model space distance between geometric entities at asserted c
onnectivities');
#62885=UNCERTAINTY_MEASURE_WITH_UNIT(LENGTH_MEASURE(0.001),#62985,
'DISTANCE_ACCURACY_VALUE',
'Maximum model space distance between geometric entities at asserted c
onnectivities');
#62917=(
GEOMETRIC_REPRESENTATION_CONTEXT(3)
GLOBAL_UNCERTAINTY_ASSIGNED_CONTEXT((#62818))
GLOBAL_UNIT_ASSIGNED_CONTEXT((#62985,#62987,#62988))
REPRESENTATION_CONTEXT('','3D')
);
#62984=(
GEOMETRIC_REPRESENTATION_CONTEXT(3)
GLOBAL_UNCERTAINTY_ASSIGNED_CONTEXT((#62885))
GLOBAL_UNIT_ASSIGNED_CONTEXT((#62985,#62987,#62988))
REPRESENTATION_CONTEXT('','3D')
);
#62985=(
LENGTH_UNIT()
NAMED_UNIT(*)
SI_UNIT(.CENTI.,.METRE.)
);
#62987=(
NAMED_UNIT(*)
PLANE_ANGLE_UNIT()
SI_UNIT($,.RADIAN.)
);
#62988=(
NAMED_UNIT(*)
SI_UNIT($,.STERADIAN.)
SOLID_ANGLE_UNIT()
);
#63020=SHAPE_DEFINITION_REPRESENTATION(#63128,#63380);
#63128=PRODUCT_DEFINITION_SHAPE('',$,#63479);
#63380=SHAPE_REPRESENTATION('',(#24649),#62917);
#63447=PRODUCT_DEFINITION_CONTEXT('part definition',#63743,'design');
#63479=PRODUCT_DEFINITION('Block','Block',#63577,#63447);
#63577=PRODUCT_DEFINITION_FORMATION('',$,#63776);
#63743=APPLICATION_CONTEXT(
'Core Data for Automotive Mechanical Design Process');
#63744=PRODUCT_CONTEXT('part definition',#63743,'mechanical');
#63776=PRODUCT('Block','Block','Block',(#63744));
#63885=COLOUR_RGB('Dark Blue',0.08,0.2,0.34);
#63886=FILL_AREA_STYLE_COLOUR('',#63885);
#63887=FILL_AREA_STYLE('',(#63886));
#63888=SURFACE_STYLE_FILL_AREA(#63887);
#63889=SURFACE_SIDE_STYLE('',(#63888));
#63890=SURFACE_STYLE_USAGE(.BOTH.,#63889);
#63891=PRESENTATION_STYLE_ASSIGNMENT((#63890));
ENDSEC;
END-ISO-10303-21;
